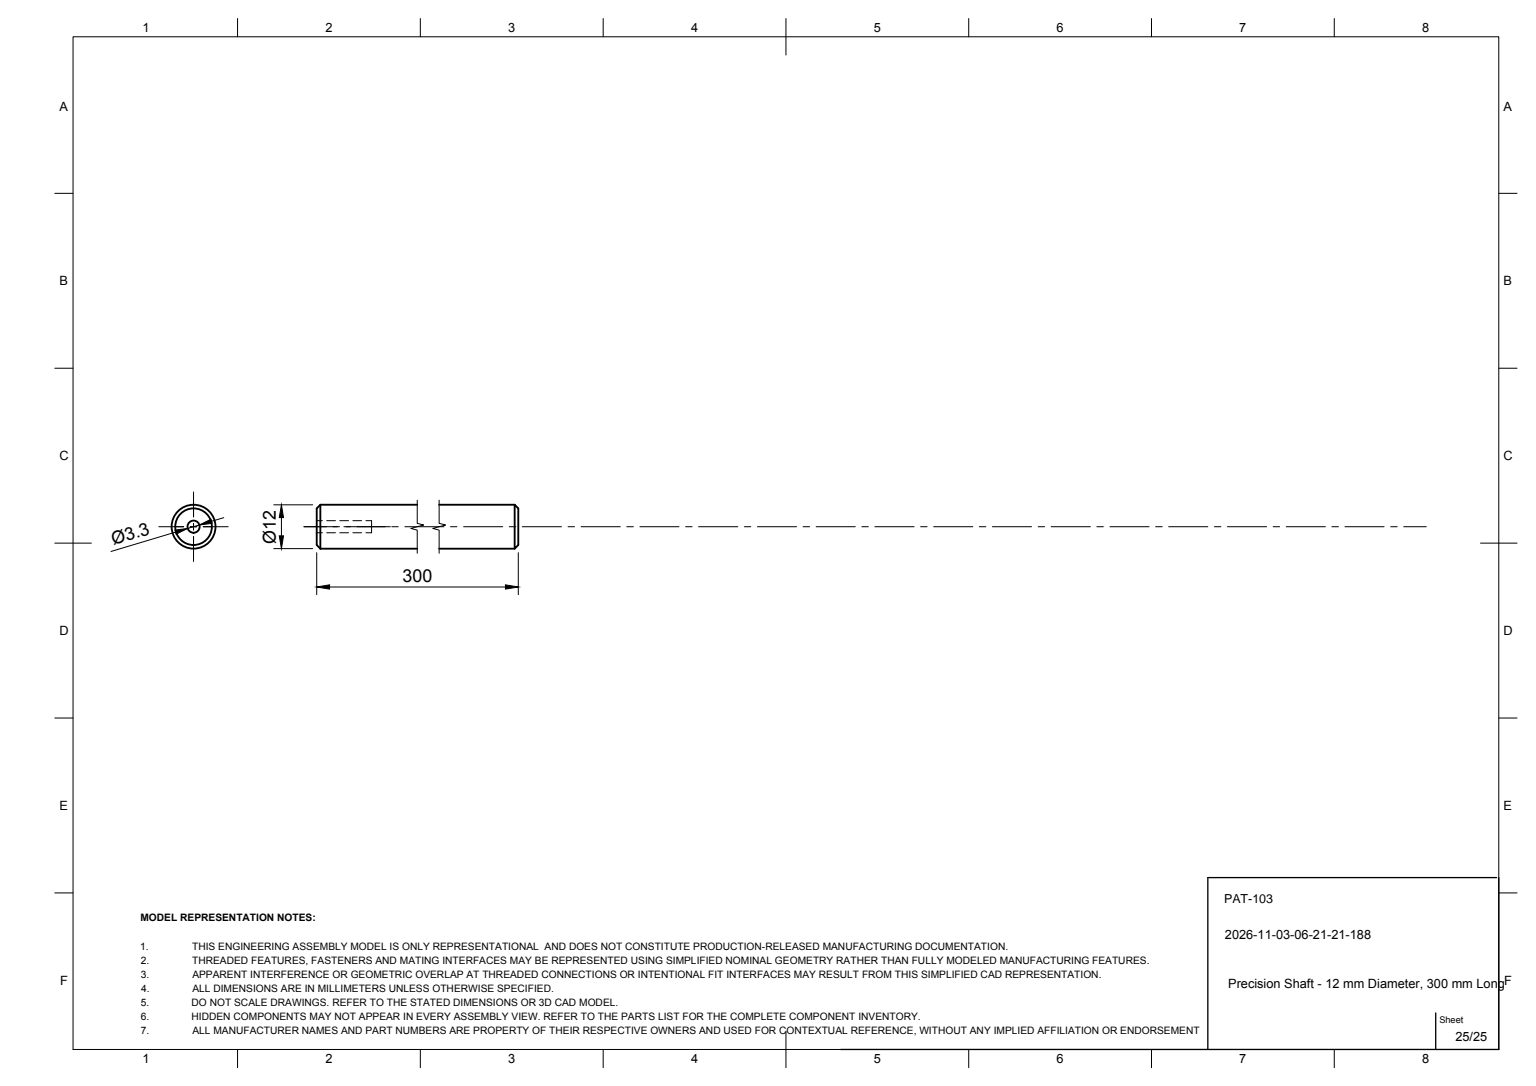
ISO-10303-21;
HEADER;
/* Generated by software containing ST-Developer
 * from STEP Tools, Inc. (www.steptools.com) 
 */

FILE_DESCRIPTION(
/* description */ ('Telescoping shaft support with lock collar'),
/* implementation_level */ '2;1');

FILE_NAME(
/* name */ 'Precision Shaft - 12 mm Diameter, 300 mm Long.step',
/* time_stamp */ '2026-10-27T10:48:51-07:00',
/* author */ (''),
/* organization */ (''),
/* preprocessor_version */ 'ST-DEVELOPER v20.2',
/* originating_system */ 'Autodesk Translation Framework v15.17.0.0',
/* authorisation */ '');

FILE_SCHEMA (('AUTOMOTIVE_DESIGN { 1 0 10303 214 3 1 1 }'));
ENDSEC;

DATA;
#10=MECHANICAL_DESIGN_GEOMETRIC_PRESENTATION_REPRESENTATION('',(#258),#7349);
#173=CONICAL_SURFACE('',#4618,0.55,0.785398163397448);
#174=CONICAL_SURFACE('',#4624,0.55,0.785398163397441);
#218=SHAPE_REPRESENTATION_RELATIONSHIP('SRR','None',#7462,#238);
#238=ADVANCED_BREP_SHAPE_REPRESENTATION('',(#277),#7346);
#258=STYLED_ITEM('',(#7627),#277);
#277=MANIFOLD_SOLID_BREP('Body1',#3982);
#356=FACE_BOUND('',#995,.T.);
#472=PLANE('',#4617);
#473=PLANE('',#4623);
#474=PLANE('',#4626);
#685=FACE_OUTER_BOUND('',#988,.T.);
#686=FACE_OUTER_BOUND('',#989,.T.);
#687=FACE_OUTER_BOUND('',#990,.T.);
#688=FACE_OUTER_BOUND('',#991,.T.);
#689=FACE_OUTER_BOUND('',#992,.T.);
#690=FACE_OUTER_BOUND('',#993,.T.);
#691=FACE_OUTER_BOUND('',#994,.T.);
#988=EDGE_LOOP('',(#3526,#3527,#3528,#3529));
#989=EDGE_LOOP('',(#3530));
#990=EDGE_LOOP('',(#3531,#3532,#3533,#3534));
#991=EDGE_LOOP('',(#3535,#3536,#3537,#3538));
#992=EDGE_LOOP('',(#3539));
#993=EDGE_LOOP('',(#3540,#3541,#3542,#3543));
#994=EDGE_LOOP('',(#3544));
#995=EDGE_LOOP('',(#3545));
#1258=LINE('',#7120,#1538);
#1259=LINE('',#7127,#1539);
#1260=LINE('',#7132,#1540);
#1261=LINE('',#7137,#1541);
#1538=VECTOR('',#5756,0.165);
#1539=VECTOR('',#5765,0.55);
#1540=VECTOR('',#5772,0.6);
#1541=VECTOR('',#5779,0.55);
#1780=CIRCLE('',#4615,0.165);
#1781=CIRCLE('',#4616,0.165);
#1782=CIRCLE('',#4619,0.6);
#1783=CIRCLE('',#4620,0.5);
#1784=CIRCLE('',#4622,0.6);
#1785=CIRCLE('',#4625,0.5);
#2091=VERTEX_POINT('',#7117);
#2092=VERTEX_POINT('',#7119);
#2093=VERTEX_POINT('',#7124);
#2094=VERTEX_POINT('',#7126);
#2095=VERTEX_POINT('',#7130);
#2096=VERTEX_POINT('',#7135);
#2575=EDGE_CURVE('',#2091,#2091,#1780,.T.);
#2576=EDGE_CURVE('',#2091,#2092,#1258,.T.);
#2577=EDGE_CURVE('',#2092,#2092,#1781,.T.);
#2578=EDGE_CURVE('',#2093,#2093,#1782,.T.);
#2579=EDGE_CURVE('',#2093,#2094,#1259,.T.);
#2580=EDGE_CURVE('',#2094,#2094,#1783,.T.);
#2581=EDGE_CURVE('',#2095,#2095,#1784,.T.);
#2582=EDGE_CURVE('',#2095,#2093,#1260,.T.);
#2583=EDGE_CURVE('',#2096,#2096,#1785,.T.);
#2584=EDGE_CURVE('',#2096,#2095,#1261,.T.);
#3526=ORIENTED_EDGE('',*,*,#2575,.F.);
#3527=ORIENTED_EDGE('',*,*,#2576,.T.);
#3528=ORIENTED_EDGE('',*,*,#2577,.F.);
#3529=ORIENTED_EDGE('',*,*,#2576,.F.);
#3530=ORIENTED_EDGE('',*,*,#2575,.T.);
#3531=ORIENTED_EDGE('',*,*,#2578,.T.);
#3532=ORIENTED_EDGE('',*,*,#2579,.T.);
#3533=ORIENTED_EDGE('',*,*,#2580,.T.);
#3534=ORIENTED_EDGE('',*,*,#2579,.F.);
#3535=ORIENTED_EDGE('',*,*,#2581,.F.);
#3536=ORIENTED_EDGE('',*,*,#2582,.T.);
#3537=ORIENTED_EDGE('',*,*,#2578,.F.);
#3538=ORIENTED_EDGE('',*,*,#2582,.F.);
#3539=ORIENTED_EDGE('',*,*,#2580,.F.);
#3540=ORIENTED_EDGE('',*,*,#2583,.T.);
#3541=ORIENTED_EDGE('',*,*,#2584,.T.);
#3542=ORIENTED_EDGE('',*,*,#2581,.T.);
#3543=ORIENTED_EDGE('',*,*,#2584,.F.);
#3544=ORIENTED_EDGE('',*,*,#2583,.F.);
#3545=ORIENTED_EDGE('',*,*,#2577,.T.);
#3733=CYLINDRICAL_SURFACE('',#4614,0.165);
#3734=CYLINDRICAL_SURFACE('',#4621,0.6);
#3928=ADVANCED_FACE('',(#685),#3733,.F.);
#3929=ADVANCED_FACE('',(#686),#472,.T.);
#3930=ADVANCED_FACE('',(#687),#173,.T.);
#3931=ADVANCED_FACE('',(#688),#3734,.T.);
#3932=ADVANCED_FACE('',(#689),#473,.F.);
#3933=ADVANCED_FACE('',(#690),#174,.T.);
#3934=ADVANCED_FACE('',(#691,#356),#474,.T.);
#3982=CLOSED_SHELL('',(#3928,#3929,#3930,#3931,#3932,#3933,#3934));
#4613=AXIS2_PLACEMENT_3D('',#7115,#5750,#5751);
#4614=AXIS2_PLACEMENT_3D('',#7116,#5752,#5753);
#4615=AXIS2_PLACEMENT_3D('',#7118,#5754,#5755);
#4616=AXIS2_PLACEMENT_3D('',#7121,#5757,#5758);
#4617=AXIS2_PLACEMENT_3D('',#7122,#5759,#5760);
#4618=AXIS2_PLACEMENT_3D('',#7123,#5761,#5762);
#4619=AXIS2_PLACEMENT_3D('',#7125,#5763,#5764);
#4620=AXIS2_PLACEMENT_3D('',#7128,#5766,#5767);
#4621=AXIS2_PLACEMENT_3D('',#7129,#5768,#5769);
#4622=AXIS2_PLACEMENT_3D('',#7131,#5770,#5771);
#4623=AXIS2_PLACEMENT_3D('',#7133,#5773,#5774);
#4624=AXIS2_PLACEMENT_3D('',#7134,#5775,#5776);
#4625=AXIS2_PLACEMENT_3D('',#7136,#5777,#5778);
#4626=AXIS2_PLACEMENT_3D('',#7138,#5780,#5781);
#5750=DIRECTION('axis',(0.,0.,1.));
#5751=DIRECTION('refdir',(1.,0.,0.));
#5752=DIRECTION('center_axis',(1.,0.,0.));
#5753=DIRECTION('ref_axis',(0.,0.,-1.));
#5754=DIRECTION('center_axis',(1.,0.,0.));
#5755=DIRECTION('ref_axis',(0.,0.,-1.));
#5756=DIRECTION('',(1.,0.,0.));
#5757=DIRECTION('center_axis',(-1.,0.,0.));
#5758=DIRECTION('ref_axis',(0.,0.,-1.));
#5759=DIRECTION('center_axis',(1.,0.,0.));
#5760=DIRECTION('ref_axis',(0.,0.,-1.));
#5761=DIRECTION('center_axis',(1.,0.,0.));
#5762=DIRECTION('ref_axis',(0.,0.,-1.));
#5763=DIRECTION('center_axis',(-1.,0.,0.));
#5764=DIRECTION('ref_axis',(0.,0.,-1.));
#5765=DIRECTION('',(-0.707106781186548,8.65956056235493E-17,-0.707106781186547));
#5766=DIRECTION('center_axis',(1.,0.,0.));
#5767=DIRECTION('ref_axis',(0.,0.,-1.));
#5768=DIRECTION('center_axis',(1.,0.,0.));
#5769=DIRECTION('ref_axis',(0.,0.,-1.));
#5770=DIRECTION('center_axis',(1.,0.,0.));
#5771=DIRECTION('ref_axis',(0.,0.,-1.));
#5772=DIRECTION('',(-1.,0.,0.));
#5773=DIRECTION('center_axis',(1.,0.,0.));
#5774=DIRECTION('ref_axis',(0.,0.,-1.));
#5775=DIRECTION('center_axis',(-1.,0.,0.));
#5776=DIRECTION('ref_axis',(0.,0.,-1.));
#5777=DIRECTION('center_axis',(-1.,0.,0.));
#5778=DIRECTION('ref_axis',(0.,0.,-1.));
#5779=DIRECTION('',(-0.707106781186553,-8.65956056235487E-17,0.707106781186542));
#5780=DIRECTION('center_axis',(1.,0.,0.));
#5781=DIRECTION('ref_axis',(0.,0.,-1.));
#7115=CARTESIAN_POINT('',(0.,0.,0.));
#7116=CARTESIAN_POINT('Origin',(28.5,0.,0.));
#7117=CARTESIAN_POINT('',(28.5,-2.02066721859313E-17,0.165));
#7118=CARTESIAN_POINT('Origin',(28.5,0.,0.));
#7119=CARTESIAN_POINT('',(30.,2.02066721859313E-17,0.165));
#7120=CARTESIAN_POINT('',(28.5,-2.02066721859313E-17,0.165));
#7121=CARTESIAN_POINT('Origin',(30.,0.,0.));
#7122=CARTESIAN_POINT('Origin',(28.5,0.,0.));
#7123=CARTESIAN_POINT('Origin',(0.05,0.,0.));
#7124=CARTESIAN_POINT('',(0.1,7.34788079488412E-17,0.6));
#7125=CARTESIAN_POINT('Origin',(0.1,0.,0.));
#7126=CARTESIAN_POINT('',(0.,-6.12323399573677E-17,0.5));
#7127=CARTESIAN_POINT('',(0.05,-6.73555739531044E-17,0.55));
#7128=CARTESIAN_POINT('Origin',(0.,0.,0.));
#7129=CARTESIAN_POINT('Origin',(0.,0.,0.));
#7130=CARTESIAN_POINT('',(29.9,-7.34788079488412E-17,0.6));
#7131=CARTESIAN_POINT('Origin',(29.9,0.,0.));
#7132=CARTESIAN_POINT('',(0.,-7.34788079488412E-17,0.6));
#7133=CARTESIAN_POINT('Origin',(0.,0.,0.));
#7134=CARTESIAN_POINT('Origin',(29.95,0.,0.));
#7135=CARTESIAN_POINT('',(30.,6.12323399573677E-17,0.5));
#7136=CARTESIAN_POINT('Origin',(30.,0.,0.));
#7137=CARTESIAN_POINT('',(29.95,-6.73555739531044E-17,0.55));
#7138=CARTESIAN_POINT('Origin',(30.,0.,0.));
#7321=UNCERTAINTY_MEASURE_WITH_UNIT(LENGTH_MEASURE(0.001),#7350,
'DISTANCE_ACCURACY_VALUE',
'Maximum model space distance between geometric entities at asserted c
onnectivities');
#7324=UNCERTAINTY_MEASURE_WITH_UNIT(LENGTH_MEASURE(0.001),#7350,
'DISTANCE_ACCURACY_VALUE',
'Maximum model space distance between geometric entities at asserted c
onnectivities');
#7346=(
GEOMETRIC_REPRESENTATION_CONTEXT(3)
GLOBAL_UNCERTAINTY_ASSIGNED_CONTEXT((#7321))
GLOBAL_UNIT_ASSIGNED_CONTEXT((#7350,#7352,#7353))
REPRESENTATION_CONTEXT('','3D')
);
#7349=(
GEOMETRIC_REPRESENTATION_CONTEXT(3)
GLOBAL_UNCERTAINTY_ASSIGNED_CONTEXT((#7324))
GLOBAL_UNIT_ASSIGNED_CONTEXT((#7350,#7352,#7353))
REPRESENTATION_CONTEXT('','3D')
);
#7350=(
LENGTH_UNIT()
NAMED_UNIT(*)
SI_UNIT(.CENTI.,.METRE.)
);
#7352=(
NAMED_UNIT(*)
PLANE_ANGLE_UNIT()
SI_UNIT($,.RADIAN.)
);
#7353=(
NAMED_UNIT(*)
SI_UNIT($,.STERADIAN.)
SOLID_ANGLE_UNIT()
);
#7375=SHAPE_DEFINITION_REPRESENTATION(#7401,#7462);
#7401=PRODUCT_DEFINITION_SHAPE('',$,#7487);
#7462=SHAPE_REPRESENTATION('',(#4613),#7346);
#7465=PRODUCT_DEFINITION_CONTEXT('part definition',#7539,'design');
#7487=PRODUCT_DEFINITION(
'Precision Shaft - 12 mm Diameter, 300 mm Long',
'Precision Shaft - 12 mm Diameter, 300 mm Long',#7511,#7465);
#7511=PRODUCT_DEFINITION_FORMATION('',$,#7562);
#7539=APPLICATION_CONTEXT(
'Core Data for Automotive Mechanical Design Process');
#7540=PRODUCT_CONTEXT('part definition',#7539,'mechanical');
#7562=PRODUCT('Precision Shaft - 12 mm Diameter, 300 mm Long',
'Precision Shaft - 12 mm Diameter, 300 mm Long',
'Precision Shaft - 12 mm Diameter, 300 mm Long',(#7540));
#7621=COLOUR_RGB('Grey',0.48,0.52,0.57);
#7622=FILL_AREA_STYLE_COLOUR('',#7621);
#7623=FILL_AREA_STYLE('',(#7622));
#7624=SURFACE_STYLE_FILL_AREA(#7623);
#7625=SURFACE_SIDE_STYLE('',(#7624));
#7626=SURFACE_STYLE_USAGE(.BOTH.,#7625);
#7627=PRESENTATION_STYLE_ASSIGNMENT((#7626));
ENDSEC;
END-ISO-10303-21;
